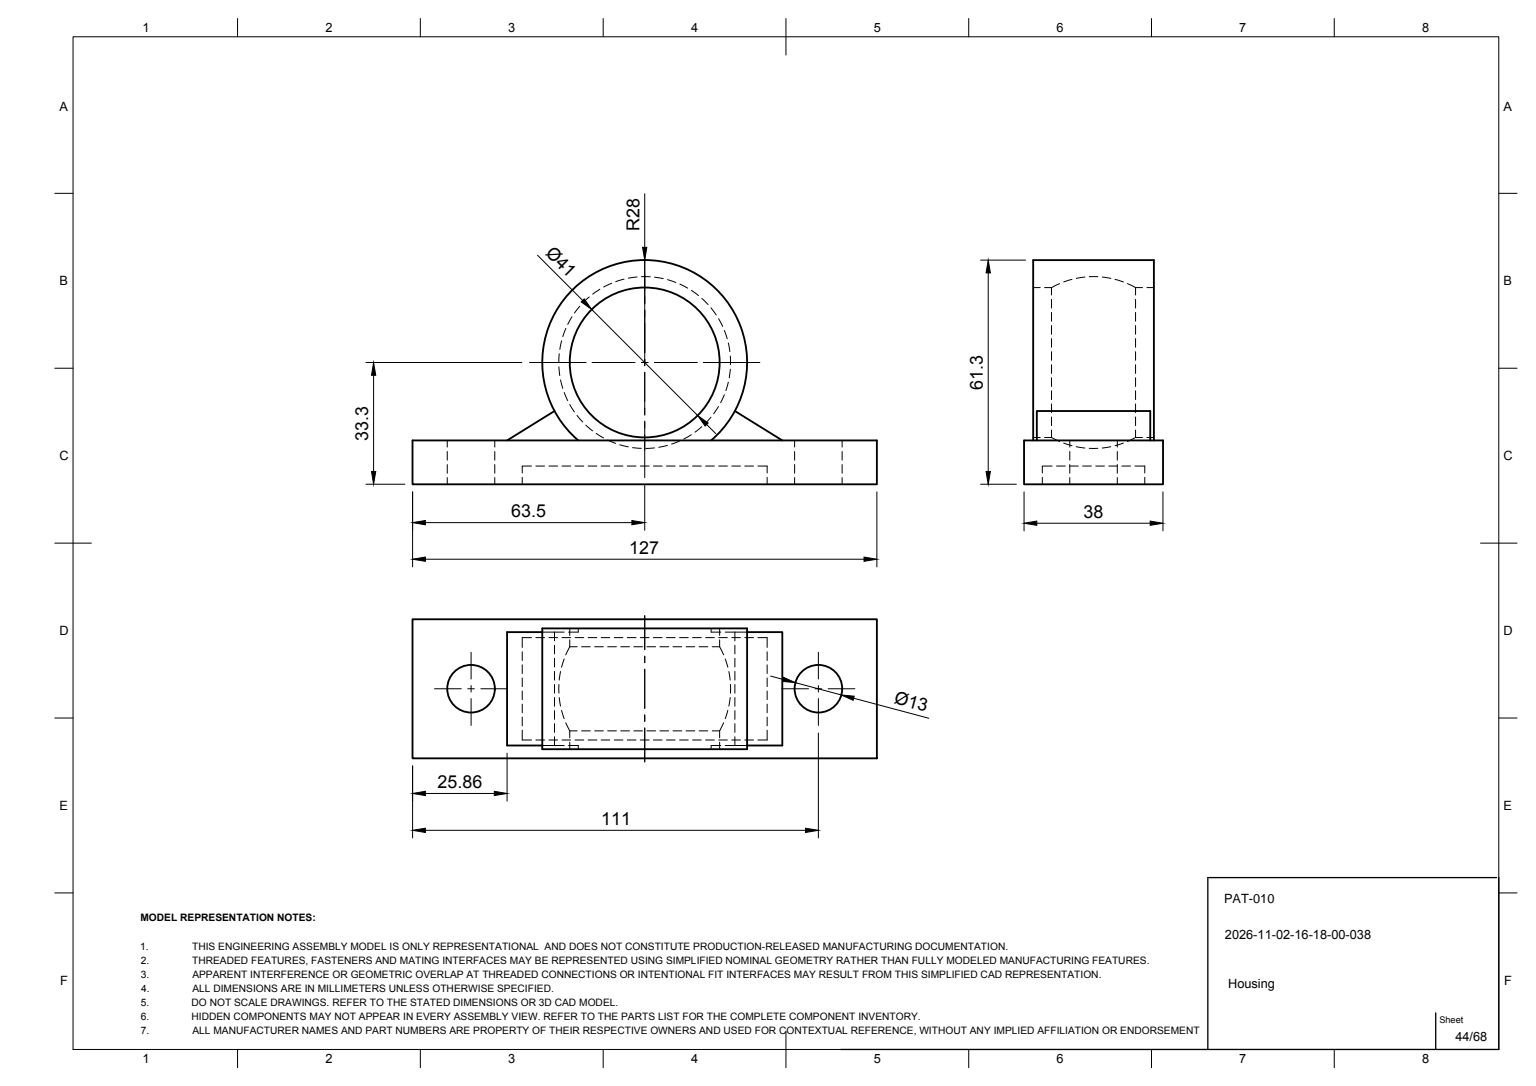
ISO-10303-21;
HEADER;
/* Generated by software containing ST-Developer
 * from STEP Tools, Inc. (www.steptools.com) 
 */

FILE_DESCRIPTION(
/* description */ ('Belt conveyor head drive unit'),
/* implementation_level */ '2;1');

FILE_NAME(
/* name */ 'Housing.step',
/* time_stamp */ '2026-10-28T03:26:19-07:00',
/* author */ (''),
/* organization */ (''),
/* preprocessor_version */ 'ST-DEVELOPER v20.2',
/* originating_system */ 'Autodesk Translation Framework v15.17.0.0',
/* authorisation */ '');

FILE_SCHEMA (('AUTOMOTIVE_DESIGN { 1 0 10303 214 3 1 1 }'));
ENDSEC;

DATA;
#10=MECHANICAL_DESIGN_GEOMETRIC_PRESENTATION_REPRESENTATION('',(#901),#27069);
#675=SPHERICAL_SURFACE('',#15515,2.35);
#748=SHAPE_REPRESENTATION_RELATIONSHIP('SRR','None',#27395,#817);
#817=ADVANCED_BREP_SHAPE_REPRESENTATION('',(#984),#27037);
#901=STYLED_ITEM('',(#27776),#984);
#984=MANIFOLD_SOLID_BREP('Body1',#13768);
#1172=FACE_BOUND('',#3033,.T.);
#1173=FACE_BOUND('',#3034,.T.);
#1174=FACE_BOUND('',#3042,.T.);
#1175=FACE_BOUND('',#3043,.T.);
#1176=FACE_BOUND('',#3044,.T.);
#1177=FACE_BOUND('',#3047,.T.);
#1178=FACE_BOUND('',#3049,.T.);
#1179=FACE_BOUND('',#3062,.T.);
#1180=FACE_BOUND('',#3063,.T.);
#1181=FACE_BOUND('',#3064,.T.);
#1493=PLANE('',#15517);
#1494=PLANE('',#15519);
#1495=PLANE('',#15521);
#1496=PLANE('',#15523);
#1497=PLANE('',#15524);
#1498=PLANE('',#15526);
#1499=PLANE('',#15527);
#1500=PLANE('',#15533);
#1501=PLANE('',#15534);
#1502=PLANE('',#15535);
#1503=PLANE('',#15536);
#1504=PLANE('',#15537);
#1505=PLANE('',#15538);
#1506=PLANE('',#15539);
#1507=PLANE('',#15544);
#1508=PLANE('',#15545);
#1509=PLANE('',#15546);
#1510=PLANE('',#15547);
#1511=PLANE('',#15548);
#2070=FACE_OUTER_BOUND('',#3030,.T.);
#2071=FACE_OUTER_BOUND('',#3031,.T.);
#2072=FACE_OUTER_BOUND('',#3032,.T.);
#2073=FACE_OUTER_BOUND('',#3035,.T.);
#2074=FACE_OUTER_BOUND('',#3036,.T.);
#2075=FACE_OUTER_BOUND('',#3037,.T.);
#2076=FACE_OUTER_BOUND('',#3038,.T.);
#2077=FACE_OUTER_BOUND('',#3039,.T.);
#2078=FACE_OUTER_BOUND('',#3040,.T.);
#2079=FACE_OUTER_BOUND('',#3041,.T.);
#2080=FACE_OUTER_BOUND('',#3045,.T.);
#2081=FACE_OUTER_BOUND('',#3046,.T.);
#2082=FACE_OUTER_BOUND('',#3048,.T.);
#2083=FACE_OUTER_BOUND('',#3050,.T.);
#2084=FACE_OUTER_BOUND('',#3051,.T.);
#2085=FACE_OUTER_BOUND('',#3052,.T.);
#2086=FACE_OUTER_BOUND('',#3053,.T.);
#2087=FACE_OUTER_BOUND('',#3054,.T.);
#2088=FACE_OUTER_BOUND('',#3055,.T.);
#2089=FACE_OUTER_BOUND('',#3056,.T.);
#2090=FACE_OUTER_BOUND('',#3057,.T.);
#2091=FACE_OUTER_BOUND('',#3058,.T.);
#2092=FACE_OUTER_BOUND('',#3059,.T.);
#2093=FACE_OUTER_BOUND('',#3060,.T.);
#2094=FACE_OUTER_BOUND('',#3061,.T.);
#3030=EDGE_LOOP('',(#10816,#10817,#10818,#10819));
#3031=EDGE_LOOP('',(#10820,#10821,#10822,#10823));
#3032=EDGE_LOOP('',(#10824,#10825));
#3033=EDGE_LOOP('',(#10826));
#3034=EDGE_LOOP('',(#10827));
#3035=EDGE_LOOP('',(#10828,#10829,#10830));
#3036=EDGE_LOOP('',(#10831,#10832,#10833));
#3037=EDGE_LOOP('',(#10834,#10835,#10836));
#3038=EDGE_LOOP('',(#10837,#10838,#10839,#10840));
#3039=EDGE_LOOP('',(#10841,#10842,#10843));
#3040=EDGE_LOOP('',(#10844,#10845,#10846,#10847));
#3041=EDGE_LOOP('',(#10848,#10849,#10850,#10851));
#3042=EDGE_LOOP('',(#10852));
#3043=EDGE_LOOP('',(#10853));
#3044=EDGE_LOOP('',(#10854,#10855,#10856,#10857,#10858,#10859,#10860,#10861,
#10862,#10863,#10864,#10865));
#3045=EDGE_LOOP('',(#10866,#10867,#10868,#10869,#10870,#10871,#10872,#10873,
#10874,#10875,#10876,#10877));
#3046=EDGE_LOOP('',(#10878,#10879));
#3047=EDGE_LOOP('',(#10880));
#3048=EDGE_LOOP('',(#10881,#10882));
#3049=EDGE_LOOP('',(#10883));
#3050=EDGE_LOOP('',(#10884,#10885,#10886,#10887));
#3051=EDGE_LOOP('',(#10888,#10889,#10890,#10891));
#3052=EDGE_LOOP('',(#10892,#10893,#10894,#10895));
#3053=EDGE_LOOP('',(#10896,#10897,#10898,#10899));
#3054=EDGE_LOOP('',(#10900,#10901,#10902,#10903));
#3055=EDGE_LOOP('',(#10904,#10905,#10906,#10907));
#3056=EDGE_LOOP('',(#10908,#10909,#10910,#10911));
#3057=EDGE_LOOP('',(#10912,#10913,#10914,#10915));
#3058=EDGE_LOOP('',(#10916,#10917,#10918,#10919));
#3059=EDGE_LOOP('',(#10920,#10921,#10922,#10923));
#3060=EDGE_LOOP('',(#10924,#10925,#10926,#10927));
#3061=EDGE_LOOP('',(#10928,#10929,#10930,#10931));
#3062=EDGE_LOOP('',(#10932,#10933,#10934,#10935));
#3063=EDGE_LOOP('',(#10936));
#3064=EDGE_LOOP('',(#10937));
#3940=LINE('',#23661,#4732);
#3941=LINE('',#23667,#4733);
#3942=LINE('',#23676,#4734);
#3943=LINE('',#23678,#4735);
#3944=LINE('',#23683,#4736);
#3945=LINE('',#23686,#4737);
#3946=LINE('',#23690,#4738);
#3947=LINE('',#23693,#4739);
#3948=LINE('',#23695,#4740);
#3949=LINE('',#23696,#4741);
#3950=LINE('',#23700,#4742);
#3951=LINE('',#23702,#4743);
#3952=LINE('',#23705,#4744);
#3953=LINE('',#23706,#4745);
#3954=LINE('',#23710,#4746);
#3955=LINE('',#23712,#4747);
#3956=LINE('',#23714,#4748);
#3957=LINE('',#23715,#4749);
#3958=LINE('',#23721,#4750);
#3959=LINE('',#23723,#4751);
#3960=LINE('',#23724,#4752);
#3961=LINE('',#23726,#4753);
#3962=LINE('',#23728,#4754);
#3963=LINE('',#23729,#4755);
#3964=LINE('',#23738,#4756);
#3965=LINE('',#23740,#4757);
#3966=LINE('',#23742,#4758);
#3967=LINE('',#23743,#4759);
#3968=LINE('',#23746,#4760);
#3969=LINE('',#23748,#4761);
#3970=LINE('',#23749,#4762);
#3971=LINE('',#23752,#4763);
#3972=LINE('',#23754,#4764);
#3973=LINE('',#23755,#4765);
#3974=LINE('',#23757,#4766);
#3975=LINE('',#23758,#4767);
#3976=LINE('',#23763,#4768);
#3977=LINE('',#23767,#4769);
#3978=LINE('',#23771,#4770);
#3979=LINE('',#23772,#4771);
#3980=LINE('',#23773,#4772);
#3981=LINE('',#23776,#4773);
#3982=LINE('',#23777,#4774);
#3983=LINE('',#23780,#4775);
#3984=LINE('',#23781,#4776);
#3985=LINE('',#23783,#4777);
#4732=VECTOR('',#18774,2.05);
#4733=VECTOR('',#18781,2.05);
#4734=VECTOR('',#18790,1.);
#4735=VECTOR('',#18791,1.);
#4736=VECTOR('',#18796,1.);
#4737=VECTOR('',#18799,1.);
#4738=VECTOR('',#18802,1.);
#4739=VECTOR('',#18805,1.);
#4740=VECTOR('',#18808,1.);
#4741=VECTOR('',#18809,1.);
#4742=VECTOR('',#18812,1.);
#4743=VECTOR('',#18813,1.);
#4744=VECTOR('',#18818,1.);
#4745=VECTOR('',#18819,1.);
#4746=VECTOR('',#18822,1.);
#4747=VECTOR('',#18823,1.);
#4748=VECTOR('',#18824,1.);
#4749=VECTOR('',#18825,1.);
#4750=VECTOR('',#18830,1.);
#4751=VECTOR('',#18831,1.);
#4752=VECTOR('',#18832,1.);
#4753=VECTOR('',#18833,1.);
#4754=VECTOR('',#18834,1.);
#4755=VECTOR('',#18835,1.);
#4756=VECTOR('',#18848,1.);
#4757=VECTOR('',#18849,1.);
#4758=VECTOR('',#18850,1.);
#4759=VECTOR('',#18851,1.);
#4760=VECTOR('',#18854,1.);
#4761=VECTOR('',#18855,1.);
#4762=VECTOR('',#18856,1.);
#4763=VECTOR('',#18859,1.);
#4764=VECTOR('',#18860,1.);
#4765=VECTOR('',#18861,1.);
#4766=VECTOR('',#18864,1.);
#4767=VECTOR('',#18865,1.);
#4768=VECTOR('',#18872,0.65);
#4769=VECTOR('',#18877,0.65);
#4770=VECTOR('',#18880,1.);
#4771=VECTOR('',#18881,1.);
#4772=VECTOR('',#18882,1.);
#4773=VECTOR('',#18885,1.);
#4774=VECTOR('',#18886,1.);
#4775=VECTOR('',#18889,1.);
#4776=VECTOR('',#18890,1.);
#4777=VECTOR('',#18893,1.);
#5537=CIRCLE('',#15510,2.05);
#5538=CIRCLE('',#15511,2.05);
#5539=CIRCLE('',#15513,2.05);
#5540=CIRCLE('',#15514,2.05);
#5541=CIRCLE('',#15516,2.35);
#5542=CIRCLE('',#15518,2.8);
#5543=CIRCLE('',#15520,2.8);
#5544=CIRCLE('',#15522,2.8);
#5545=CIRCLE('',#15525,2.8);
#5546=CIRCLE('',#15528,0.65);
#5547=CIRCLE('',#15529,0.65);
#5548=CIRCLE('',#15531,2.8);
#5549=CIRCLE('',#15532,2.8);
#5550=CIRCLE('',#15541,0.65);
#5551=CIRCLE('',#15543,0.65);
#6587=VERTEX_POINT('',#23658);
#6588=VERTEX_POINT('',#23660);
#6589=VERTEX_POINT('',#23664);
#6590=VERTEX_POINT('',#23666);
#6591=VERTEX_POINT('',#23670);
#6592=VERTEX_POINT('',#23671);
#6593=VERTEX_POINT('',#23674);
#6594=VERTEX_POINT('',#23675);
#6595=VERTEX_POINT('',#23677);
#6596=VERTEX_POINT('',#23681);
#6597=VERTEX_POINT('',#23682);
#6598=VERTEX_POINT('',#23684);
#6599=VERTEX_POINT('',#23688);
#6600=VERTEX_POINT('',#23689);
#6601=VERTEX_POINT('',#23691);
#6602=VERTEX_POINT('',#23698);
#6603=VERTEX_POINT('',#23699);
#6604=VERTEX_POINT('',#23701);
#6605=VERTEX_POINT('',#23708);
#6606=VERTEX_POINT('',#23709);
#6607=VERTEX_POINT('',#23711);
#6608=VERTEX_POINT('',#23713);
#6609=VERTEX_POINT('',#23716);
#6610=VERTEX_POINT('',#23718);
#6611=VERTEX_POINT('',#23720);
#6612=VERTEX_POINT('',#23722);
#6613=VERTEX_POINT('',#23725);
#6614=VERTEX_POINT('',#23727);
#6615=VERTEX_POINT('',#23736);
#6616=VERTEX_POINT('',#23737);
#6617=VERTEX_POINT('',#23739);
#6618=VERTEX_POINT('',#23741);
#6619=VERTEX_POINT('',#23745);
#6620=VERTEX_POINT('',#23747);
#6621=VERTEX_POINT('',#23751);
#6622=VERTEX_POINT('',#23753);
#6623=VERTEX_POINT('',#23761);
#6624=VERTEX_POINT('',#23765);
#6625=VERTEX_POINT('',#23769);
#6626=VERTEX_POINT('',#23770);
#6627=VERTEX_POINT('',#23775);
#6628=VERTEX_POINT('',#23779);
#8100=EDGE_CURVE('',#6587,#6587,#5537,.T.);
#8101=EDGE_CURVE('',#6587,#6588,#3940,.T.);
#8102=EDGE_CURVE('',#6588,#6588,#5538,.T.);
#8103=EDGE_CURVE('',#6589,#6589,#5539,.T.);
#8104=EDGE_CURVE('',#6589,#6590,#3941,.T.);
#8105=EDGE_CURVE('',#6590,#6590,#5540,.T.);
#8106=EDGE_CURVE('',#6591,#6592,#5541,.T.);
#8107=EDGE_CURVE('',#6593,#6594,#3942,.T.);
#8108=EDGE_CURVE('',#6593,#6595,#3943,.T.);
#8109=EDGE_CURVE('',#6594,#6595,#5542,.T.);
#8110=EDGE_CURVE('',#6596,#6597,#3944,.T.);
#8111=EDGE_CURVE('',#6598,#6596,#5543,.T.);
#8112=EDGE_CURVE('',#6598,#6597,#3945,.T.);
#8113=EDGE_CURVE('',#6599,#6600,#3946,.T.);
#8114=EDGE_CURVE('',#6601,#6599,#5544,.T.);
#8115=EDGE_CURVE('',#6601,#6600,#3947,.T.);
#8116=EDGE_CURVE('',#6600,#6593,#3948,.T.);
#8117=EDGE_CURVE('',#6595,#6601,#3949,.T.);
#8118=EDGE_CURVE('',#6602,#6603,#3950,.T.);
#8119=EDGE_CURVE('',#6602,#6604,#3951,.T.);
#8120=EDGE_CURVE('',#6603,#6604,#5545,.T.);
#8121=EDGE_CURVE('',#6597,#6602,#3952,.T.);
#8122=EDGE_CURVE('',#6604,#6598,#3953,.T.);
#8123=EDGE_CURVE('',#6605,#6606,#3954,.T.);
#8124=EDGE_CURVE('',#6606,#6607,#3955,.T.);
#8125=EDGE_CURVE('',#6607,#6608,#3956,.T.);
#8126=EDGE_CURVE('',#6608,#6605,#3957,.T.);
#8127=EDGE_CURVE('',#6609,#6609,#5546,.T.);
#8128=EDGE_CURVE('',#6610,#6610,#5547,.T.);
#8129=EDGE_CURVE('',#6603,#6611,#3958,.T.);
#8130=EDGE_CURVE('',#6611,#6612,#3959,.T.);
#8131=EDGE_CURVE('',#6612,#6599,#3960,.T.);
#8132=EDGE_CURVE('',#6594,#6613,#3961,.T.);
#8133=EDGE_CURVE('',#6613,#6614,#3962,.T.);
#8134=EDGE_CURVE('',#6614,#6596,#3963,.T.);
#8135=EDGE_CURVE('',#6613,#6614,#5548,.T.);
#8136=EDGE_CURVE('',#6611,#6612,#5549,.T.);
#8137=EDGE_CURVE('',#6615,#6616,#3964,.T.);
#8138=EDGE_CURVE('',#6615,#6617,#3965,.T.);
#8139=EDGE_CURVE('',#6617,#6618,#3966,.T.);
#8140=EDGE_CURVE('',#6616,#6618,#3967,.T.);
#8141=EDGE_CURVE('',#6619,#6615,#3968,.T.);
#8142=EDGE_CURVE('',#6619,#6620,#3969,.T.);
#8143=EDGE_CURVE('',#6620,#6617,#3970,.T.);
#8144=EDGE_CURVE('',#6621,#6619,#3971,.T.);
#8145=EDGE_CURVE('',#6621,#6622,#3972,.T.);
#8146=EDGE_CURVE('',#6622,#6620,#3973,.T.);
#8147=EDGE_CURVE('',#6616,#6621,#3974,.T.);
#8148=EDGE_CURVE('',#6618,#6622,#3975,.T.);
#8149=EDGE_CURVE('',#6623,#6623,#5550,.T.);
#8150=EDGE_CURVE('',#6623,#6610,#3976,.T.);
#8151=EDGE_CURVE('',#6624,#6624,#5551,.T.);
#8152=EDGE_CURVE('',#6624,#6609,#3977,.T.);
#8153=EDGE_CURVE('',#6625,#6626,#3978,.T.);
#8154=EDGE_CURVE('',#6626,#6605,#3979,.T.);
#8155=EDGE_CURVE('',#6625,#6608,#3980,.T.);
#8156=EDGE_CURVE('',#6627,#6625,#3981,.T.);
#8157=EDGE_CURVE('',#6627,#6607,#3982,.T.);
#8158=EDGE_CURVE('',#6628,#6627,#3983,.T.);
#8159=EDGE_CURVE('',#6628,#6606,#3984,.T.);
#8160=EDGE_CURVE('',#6626,#6628,#3985,.T.);
#10816=ORIENTED_EDGE('',*,*,#8100,.F.);
#10817=ORIENTED_EDGE('',*,*,#8101,.T.);
#10818=ORIENTED_EDGE('',*,*,#8102,.F.);
#10819=ORIENTED_EDGE('',*,*,#8101,.F.);
#10820=ORIENTED_EDGE('',*,*,#8103,.F.);
#10821=ORIENTED_EDGE('',*,*,#8104,.T.);
#10822=ORIENTED_EDGE('',*,*,#8105,.F.);
#10823=ORIENTED_EDGE('',*,*,#8104,.F.);
#10824=ORIENTED_EDGE('',*,*,#8106,.T.);
#10825=ORIENTED_EDGE('',*,*,#8106,.F.);
#10826=ORIENTED_EDGE('',*,*,#8103,.T.);
#10827=ORIENTED_EDGE('',*,*,#8102,.T.);
#10828=ORIENTED_EDGE('',*,*,#8107,.F.);
#10829=ORIENTED_EDGE('',*,*,#8108,.T.);
#10830=ORIENTED_EDGE('',*,*,#8109,.F.);
#10831=ORIENTED_EDGE('',*,*,#8110,.F.);
#10832=ORIENTED_EDGE('',*,*,#8111,.F.);
#10833=ORIENTED_EDGE('',*,*,#8112,.T.);
#10834=ORIENTED_EDGE('',*,*,#8113,.F.);
#10835=ORIENTED_EDGE('',*,*,#8114,.F.);
#10836=ORIENTED_EDGE('',*,*,#8115,.T.);
#10837=ORIENTED_EDGE('',*,*,#8116,.F.);
#10838=ORIENTED_EDGE('',*,*,#8115,.F.);
#10839=ORIENTED_EDGE('',*,*,#8117,.F.);
#10840=ORIENTED_EDGE('',*,*,#8108,.F.);
#10841=ORIENTED_EDGE('',*,*,#8118,.F.);
#10842=ORIENTED_EDGE('',*,*,#8119,.T.);
#10843=ORIENTED_EDGE('',*,*,#8120,.F.);
#10844=ORIENTED_EDGE('',*,*,#8121,.F.);
#10845=ORIENTED_EDGE('',*,*,#8112,.F.);
#10846=ORIENTED_EDGE('',*,*,#8122,.F.);
#10847=ORIENTED_EDGE('',*,*,#8119,.F.);
#10848=ORIENTED_EDGE('',*,*,#8123,.T.);
#10849=ORIENTED_EDGE('',*,*,#8124,.T.);
#10850=ORIENTED_EDGE('',*,*,#8125,.T.);
#10851=ORIENTED_EDGE('',*,*,#8126,.T.);
#10852=ORIENTED_EDGE('',*,*,#8127,.T.);
#10853=ORIENTED_EDGE('',*,*,#8128,.T.);
#10854=ORIENTED_EDGE('',*,*,#8110,.T.);
#10855=ORIENTED_EDGE('',*,*,#8121,.T.);
#10856=ORIENTED_EDGE('',*,*,#8118,.T.);
#10857=ORIENTED_EDGE('',*,*,#8129,.T.);
#10858=ORIENTED_EDGE('',*,*,#8130,.T.);
#10859=ORIENTED_EDGE('',*,*,#8131,.T.);
#10860=ORIENTED_EDGE('',*,*,#8113,.T.);
#10861=ORIENTED_EDGE('',*,*,#8116,.T.);
#10862=ORIENTED_EDGE('',*,*,#8107,.T.);
#10863=ORIENTED_EDGE('',*,*,#8132,.T.);
#10864=ORIENTED_EDGE('',*,*,#8133,.T.);
#10865=ORIENTED_EDGE('',*,*,#8134,.T.);
#10866=ORIENTED_EDGE('',*,*,#8111,.T.);
#10867=ORIENTED_EDGE('',*,*,#8134,.F.);
#10868=ORIENTED_EDGE('',*,*,#8135,.F.);
#10869=ORIENTED_EDGE('',*,*,#8132,.F.);
#10870=ORIENTED_EDGE('',*,*,#8109,.T.);
#10871=ORIENTED_EDGE('',*,*,#8117,.T.);
#10872=ORIENTED_EDGE('',*,*,#8114,.T.);
#10873=ORIENTED_EDGE('',*,*,#8131,.F.);
#10874=ORIENTED_EDGE('',*,*,#8136,.F.);
#10875=ORIENTED_EDGE('',*,*,#8129,.F.);
#10876=ORIENTED_EDGE('',*,*,#8120,.T.);
#10877=ORIENTED_EDGE('',*,*,#8122,.T.);
#10878=ORIENTED_EDGE('',*,*,#8130,.F.);
#10879=ORIENTED_EDGE('',*,*,#8136,.T.);
#10880=ORIENTED_EDGE('',*,*,#8100,.T.);
#10881=ORIENTED_EDGE('',*,*,#8133,.F.);
#10882=ORIENTED_EDGE('',*,*,#8135,.T.);
#10883=ORIENTED_EDGE('',*,*,#8105,.T.);
#10884=ORIENTED_EDGE('',*,*,#8137,.F.);
#10885=ORIENTED_EDGE('',*,*,#8138,.T.);
#10886=ORIENTED_EDGE('',*,*,#8139,.T.);
#10887=ORIENTED_EDGE('',*,*,#8140,.F.);
#10888=ORIENTED_EDGE('',*,*,#8141,.F.);
#10889=ORIENTED_EDGE('',*,*,#8142,.T.);
#10890=ORIENTED_EDGE('',*,*,#8143,.T.);
#10891=ORIENTED_EDGE('',*,*,#8138,.F.);
#10892=ORIENTED_EDGE('',*,*,#8144,.F.);
#10893=ORIENTED_EDGE('',*,*,#8145,.T.);
#10894=ORIENTED_EDGE('',*,*,#8146,.T.);
#10895=ORIENTED_EDGE('',*,*,#8142,.F.);
#10896=ORIENTED_EDGE('',*,*,#8147,.F.);
#10897=ORIENTED_EDGE('',*,*,#8140,.T.);
#10898=ORIENTED_EDGE('',*,*,#8148,.T.);
#10899=ORIENTED_EDGE('',*,*,#8145,.F.);
#10900=ORIENTED_EDGE('',*,*,#8148,.F.);
#10901=ORIENTED_EDGE('',*,*,#8139,.F.);
#10902=ORIENTED_EDGE('',*,*,#8143,.F.);
#10903=ORIENTED_EDGE('',*,*,#8146,.F.);
#10904=ORIENTED_EDGE('',*,*,#8149,.F.);
#10905=ORIENTED_EDGE('',*,*,#8150,.T.);
#10906=ORIENTED_EDGE('',*,*,#8128,.F.);
#10907=ORIENTED_EDGE('',*,*,#8150,.F.);
#10908=ORIENTED_EDGE('',*,*,#8151,.F.);
#10909=ORIENTED_EDGE('',*,*,#8152,.T.);
#10910=ORIENTED_EDGE('',*,*,#8127,.F.);
#10911=ORIENTED_EDGE('',*,*,#8152,.F.);
#10912=ORIENTED_EDGE('',*,*,#8153,.T.);
#10913=ORIENTED_EDGE('',*,*,#8154,.T.);
#10914=ORIENTED_EDGE('',*,*,#8126,.F.);
#10915=ORIENTED_EDGE('',*,*,#8155,.F.);
#10916=ORIENTED_EDGE('',*,*,#8156,.T.);
#10917=ORIENTED_EDGE('',*,*,#8155,.T.);
#10918=ORIENTED_EDGE('',*,*,#8125,.F.);
#10919=ORIENTED_EDGE('',*,*,#8157,.F.);
#10920=ORIENTED_EDGE('',*,*,#8158,.T.);
#10921=ORIENTED_EDGE('',*,*,#8157,.T.);
#10922=ORIENTED_EDGE('',*,*,#8124,.F.);
#10923=ORIENTED_EDGE('',*,*,#8159,.F.);
#10924=ORIENTED_EDGE('',*,*,#8160,.T.);
#10925=ORIENTED_EDGE('',*,*,#8159,.T.);
#10926=ORIENTED_EDGE('',*,*,#8123,.F.);
#10927=ORIENTED_EDGE('',*,*,#8154,.F.);
#10928=ORIENTED_EDGE('',*,*,#8160,.F.);
#10929=ORIENTED_EDGE('',*,*,#8153,.F.);
#10930=ORIENTED_EDGE('',*,*,#8156,.F.);
#10931=ORIENTED_EDGE('',*,*,#8158,.F.);
#10932=ORIENTED_EDGE('',*,*,#8137,.T.);
#10933=ORIENTED_EDGE('',*,*,#8147,.T.);
#10934=ORIENTED_EDGE('',*,*,#8144,.T.);
#10935=ORIENTED_EDGE('',*,*,#8141,.T.);
#10936=ORIENTED_EDGE('',*,*,#8149,.T.);
#10937=ORIENTED_EDGE('',*,*,#8151,.T.);
#12703=CYLINDRICAL_SURFACE('',#15509,2.05);
#12704=CYLINDRICAL_SURFACE('',#15512,2.05);
#12705=CYLINDRICAL_SURFACE('',#15530,2.8);
#12706=CYLINDRICAL_SURFACE('',#15540,0.65);
#12707=CYLINDRICAL_SURFACE('',#15542,0.65);
#13349=ADVANCED_FACE('',(#2070),#12703,.F.);
#13350=ADVANCED_FACE('',(#2071),#12704,.F.);
#13351=ADVANCED_FACE('',(#2072,#1172,#1173),#675,.F.);
#13352=ADVANCED_FACE('',(#2073),#1493,.T.);
#13353=ADVANCED_FACE('',(#2074),#1494,.T.);
#13354=ADVANCED_FACE('',(#2075),#1495,.T.);
#13355=ADVANCED_FACE('',(#2076),#1496,.T.);
#13356=ADVANCED_FACE('',(#2077),#1497,.T.);
#13357=ADVANCED_FACE('',(#2078),#1498,.T.);
#13358=ADVANCED_FACE('',(#2079,#1174,#1175,#1176),#1499,.T.);
#13359=ADVANCED_FACE('',(#2080),#12705,.T.);
#13360=ADVANCED_FACE('',(#2081,#1177),#1500,.F.);
#13361=ADVANCED_FACE('',(#2082,#1178),#1501,.T.);
#13362=ADVANCED_FACE('',(#2083),#1502,.F.);
#13363=ADVANCED_FACE('',(#2084),#1503,.F.);
#13364=ADVANCED_FACE('',(#2085),#1504,.F.);
#13365=ADVANCED_FACE('',(#2086),#1505,.F.);
#13366=ADVANCED_FACE('',(#2087),#1506,.F.);
#13367=ADVANCED_FACE('',(#2088),#12706,.F.);
#13368=ADVANCED_FACE('',(#2089),#12707,.F.);
#13369=ADVANCED_FACE('',(#2090),#1507,.T.);
#13370=ADVANCED_FACE('',(#2091),#1508,.T.);
#13371=ADVANCED_FACE('',(#2092),#1509,.T.);
#13372=ADVANCED_FACE('',(#2093),#1510,.T.);
#13373=ADVANCED_FACE('',(#2094,#1179,#1180,#1181),#1511,.F.);
#13768=CLOSED_SHELL('',(#13349,#13350,#13351,#13352,#13353,#13354,#13355,
#13356,#13357,#13358,#13359,#13360,#13361,#13362,#13363,#13364,#13365,#13366,
#13367,#13368,#13369,#13370,#13371,#13372,#13373));
#15508=AXIS2_PLACEMENT_3D('',#23656,#18768,#18769);
#15509=AXIS2_PLACEMENT_3D('',#23657,#18770,#18771);
#15510=AXIS2_PLACEMENT_3D('',#23659,#18772,#18773);
#15511=AXIS2_PLACEMENT_3D('',#23662,#18775,#18776);
#15512=AXIS2_PLACEMENT_3D('',#23663,#18777,#18778);
#15513=AXIS2_PLACEMENT_3D('',#23665,#18779,#18780);
#15514=AXIS2_PLACEMENT_3D('',#23668,#18782,#18783);
#15515=AXIS2_PLACEMENT_3D('',#23669,#18784,#18785);
#15516=AXIS2_PLACEMENT_3D('',#23672,#18786,#18787);
#15517=AXIS2_PLACEMENT_3D('',#23673,#18788,#18789);
#15518=AXIS2_PLACEMENT_3D('',#23679,#18792,#18793);
#15519=AXIS2_PLACEMENT_3D('',#23680,#18794,#18795);
#15520=AXIS2_PLACEMENT_3D('',#23685,#18797,#18798);
#15521=AXIS2_PLACEMENT_3D('',#23687,#18800,#18801);
#15522=AXIS2_PLACEMENT_3D('',#23692,#18803,#18804);
#15523=AXIS2_PLACEMENT_3D('',#23694,#18806,#18807);
#15524=AXIS2_PLACEMENT_3D('',#23697,#18810,#18811);
#15525=AXIS2_PLACEMENT_3D('',#23703,#18814,#18815);
#15526=AXIS2_PLACEMENT_3D('',#23704,#18816,#18817);
#15527=AXIS2_PLACEMENT_3D('',#23707,#18820,#18821);
#15528=AXIS2_PLACEMENT_3D('',#23717,#18826,#18827);
#15529=AXIS2_PLACEMENT_3D('',#23719,#18828,#18829);
#15530=AXIS2_PLACEMENT_3D('',#23730,#18836,#18837);
#15531=AXIS2_PLACEMENT_3D('',#23731,#18838,#18839);
#15532=AXIS2_PLACEMENT_3D('',#23732,#18840,#18841);
#15533=AXIS2_PLACEMENT_3D('',#23733,#18842,#18843);
#15534=AXIS2_PLACEMENT_3D('',#23734,#18844,#18845);
#15535=AXIS2_PLACEMENT_3D('',#23735,#18846,#18847);
#15536=AXIS2_PLACEMENT_3D('',#23744,#18852,#18853);
#15537=AXIS2_PLACEMENT_3D('',#23750,#18857,#18858);
#15538=AXIS2_PLACEMENT_3D('',#23756,#18862,#18863);
#15539=AXIS2_PLACEMENT_3D('',#23759,#18866,#18867);
#15540=AXIS2_PLACEMENT_3D('',#23760,#18868,#18869);
#15541=AXIS2_PLACEMENT_3D('',#23762,#18870,#18871);
#15542=AXIS2_PLACEMENT_3D('',#23764,#18873,#18874);
#15543=AXIS2_PLACEMENT_3D('',#23766,#18875,#18876);
#15544=AXIS2_PLACEMENT_3D('',#23768,#18878,#18879);
#15545=AXIS2_PLACEMENT_3D('',#23774,#18883,#18884);
#15546=AXIS2_PLACEMENT_3D('',#23778,#18887,#18888);
#15547=AXIS2_PLACEMENT_3D('',#23782,#18891,#18892);
#15548=AXIS2_PLACEMENT_3D('',#23784,#18894,#18895);
#18768=DIRECTION('axis',(0.,0.,1.));
#18769=DIRECTION('refdir',(1.,0.,0.));
#18770=DIRECTION('center_axis',(0.,1.,0.));
#18771=DIRECTION('ref_axis',(1.,0.,0.));
#18772=DIRECTION('center_axis',(0.,1.,0.));
#18773=DIRECTION('ref_axis',(1.,0.,0.));
#18774=DIRECTION('',(0.,1.,0.));
#18775=DIRECTION('center_axis',(0.,-1.,0.));
#18776=DIRECTION('ref_axis',(1.,0.,0.));
#18777=DIRECTION('center_axis',(0.,1.,0.));
#18778=DIRECTION('ref_axis',(1.,0.,0.));
#18779=DIRECTION('center_axis',(0.,1.,0.));
#18780=DIRECTION('ref_axis',(1.,0.,0.));
#18781=DIRECTION('',(0.,1.,0.));
#18782=DIRECTION('center_axis',(0.,-1.,0.));
#18783=DIRECTION('ref_axis',(1.,0.,0.));
#18784=DIRECTION('center_axis',(6.12323399573677E-17,0.,1.));
#18785=DIRECTION('ref_axis',(1.,0.,0.));
#18786=DIRECTION('center_axis',(-1.22464679914735E-16,1.,0.));
#18787=DIRECTION('ref_axis',(-1.,-1.22464679914735E-16,0.));
#18788=DIRECTION('center_axis',(0.,1.,0.));
#18789=DIRECTION('ref_axis',(0.,0.,1.));
#18790=DIRECTION('',(1.,0.,0.));
#18791=DIRECTION('',(0.850265146687862,0.,0.526354614616295));
#18792=DIRECTION('center_axis',(0.,1.,0.));
#18793=DIRECTION('ref_axis',(1.,0.,0.));
#18794=DIRECTION('center_axis',(0.,1.,0.));
#18795=DIRECTION('ref_axis',(0.,0.,1.));
#18796=DIRECTION('',(1.,0.,0.));
#18797=DIRECTION('center_axis',(0.,1.,0.));
#18798=DIRECTION('ref_axis',(1.,0.,0.));
#18799=DIRECTION('',(0.850265146687862,0.,-0.526354614616295));
#18800=DIRECTION('center_axis',(0.,-1.,0.));
#18801=DIRECTION('ref_axis',(0.,0.,-1.));
#18802=DIRECTION('',(-1.,0.,0.));
#18803=DIRECTION('center_axis',(0.,-1.,0.));
#18804=DIRECTION('ref_axis',(1.,0.,0.));
#18805=DIRECTION('',(-0.850265146687862,0.,-0.526354614616295));
#18806=DIRECTION('center_axis',(-0.526354614616295,0.,0.850265146687862));
#18807=DIRECTION('ref_axis',(0.850265146687862,0.,0.526354614616295));
#18808=DIRECTION('',(0.,1.,0.));
#18809=DIRECTION('',(0.,-1.,0.));
#18810=DIRECTION('center_axis',(0.,-1.,0.));
#18811=DIRECTION('ref_axis',(0.,0.,-1.));
#18812=DIRECTION('',(-1.,0.,0.));
#18813=DIRECTION('',(-0.850265146687862,0.,0.526354614616295));
#18814=DIRECTION('center_axis',(0.,-1.,0.));
#18815=DIRECTION('ref_axis',(1.,0.,0.));
#18816=DIRECTION('center_axis',(0.526354614616295,0.,0.850265146687862));
#18817=DIRECTION('ref_axis',(0.850265146687862,0.,-0.526354614616295));
#18818=DIRECTION('',(0.,-1.,0.));
#18819=DIRECTION('',(0.,1.,0.));
#18820=DIRECTION('center_axis',(0.,0.,1.));
#18821=DIRECTION('ref_axis',(1.,0.,0.));
#18822=DIRECTION('',(0.,-1.,0.));
#18823=DIRECTION('',(1.,0.,0.));
#18824=DIRECTION('',(0.,1.,0.));
#18825=DIRECTION('',(-1.,0.,0.));
#18826=DIRECTION('center_axis',(0.,0.,-1.));
#18827=DIRECTION('ref_axis',(1.,0.,0.));
#18828=DIRECTION('center_axis',(0.,0.,-1.));
#18829=DIRECTION('ref_axis',(1.,0.,0.));
#18830=DIRECTION('',(0.,-1.,0.));
#18831=DIRECTION('',(-1.,0.,0.));
#18832=DIRECTION('',(0.,1.,0.));
#18833=DIRECTION('',(0.,1.,0.));
#18834=DIRECTION('',(1.,0.,0.));
#18835=DIRECTION('',(0.,-1.,0.));
#18836=DIRECTION('center_axis',(0.,1.,0.));
#18837=DIRECTION('ref_axis',(6.12323399573677E-17,0.,1.));
#18838=DIRECTION('center_axis',(0.,1.,0.));
#18839=DIRECTION('ref_axis',(1.,0.,0.));
#18840=DIRECTION('center_axis',(0.,-1.,0.));
#18841=DIRECTION('ref_axis',(1.,0.,0.));
#18842=DIRECTION('center_axis',(0.,1.,0.));
#18843=DIRECTION('ref_axis',(1.,0.,0.));
#18844=DIRECTION('center_axis',(0.,1.,0.));
#18845=DIRECTION('ref_axis',(1.,0.,0.));
#18846=DIRECTION('center_axis',(0.,1.,0.));
#18847=DIRECTION('ref_axis',(-1.,0.,0.));
#18848=DIRECTION('',(-1.,0.,0.));
#18849=DIRECTION('',(0.,0.,1.));
#18850=DIRECTION('',(-1.,0.,0.));
#18851=DIRECTION('',(0.,0.,1.));
#18852=DIRECTION('center_axis',(1.,0.,0.));
#18853=DIRECTION('ref_axis',(0.,1.,0.));
#18854=DIRECTION('',(0.,1.,0.));
#18855=DIRECTION('',(0.,0.,1.));
#18856=DIRECTION('',(0.,1.,0.));
#18857=DIRECTION('center_axis',(0.,-1.,0.));
#18858=DIRECTION('ref_axis',(1.,0.,0.));
#18859=DIRECTION('',(1.,0.,0.));
#18860=DIRECTION('',(0.,0.,1.));
#18861=DIRECTION('',(1.,0.,0.));
#18862=DIRECTION('center_axis',(-1.,0.,0.));
#18863=DIRECTION('ref_axis',(0.,-1.,0.));
#18864=DIRECTION('',(0.,-1.,0.));
#18865=DIRECTION('',(0.,-1.,0.));
#18866=DIRECTION('center_axis',(0.,0.,1.));
#18867=DIRECTION('ref_axis',(1.,0.,0.));
#18868=DIRECTION('center_axis',(0.,0.,1.));
#18869=DIRECTION('ref_axis',(1.,0.,0.));
#18870=DIRECTION('center_axis',(0.,0.,1.));
#18871=DIRECTION('ref_axis',(1.,0.,0.));
#18872=DIRECTION('',(0.,0.,1.));
#18873=DIRECTION('center_axis',(0.,0.,1.));
#18874=DIRECTION('ref_axis',(1.,0.,0.));
#18875=DIRECTION('center_axis',(0.,0.,1.));
#18876=DIRECTION('ref_axis',(1.,0.,0.));
#18877=DIRECTION('',(0.,0.,1.));
#18878=DIRECTION('center_axis',(0.,1.,0.));
#18879=DIRECTION('ref_axis',(-1.,0.,0.));
#18880=DIRECTION('',(-1.,0.,0.));
#18881=DIRECTION('',(0.,0.,1.));
#18882=DIRECTION('',(0.,0.,1.));
#18883=DIRECTION('center_axis',(1.,0.,0.));
#18884=DIRECTION('ref_axis',(0.,1.,0.));
#18885=DIRECTION('',(0.,1.,0.));
#18886=DIRECTION('',(0.,0.,1.));
#18887=DIRECTION('center_axis',(0.,-1.,0.));
#18888=DIRECTION('ref_axis',(1.,0.,0.));
#18889=DIRECTION('',(1.,0.,0.));
#18890=DIRECTION('',(0.,0.,1.));
#18891=DIRECTION('center_axis',(-1.,0.,0.));
#18892=DIRECTION('ref_axis',(0.,-1.,0.));
#18893=DIRECTION('',(0.,-1.,0.));
#18894=DIRECTION('center_axis',(0.,0.,1.));
#18895=DIRECTION('ref_axis',(1.,0.,0.));
#23656=CARTESIAN_POINT('',(0.,0.,0.));
#23657=CARTESIAN_POINT('Origin',(0.,0.,0.));
#23658=CARTESIAN_POINT('',(-2.05,-1.65,2.51052593825207E-16));
#23659=CARTESIAN_POINT('Origin',(0.,-1.65,0.));
#23660=CARTESIAN_POINT('',(-2.05,-1.14891252930761,-2.51052593825207E-16));
#23661=CARTESIAN_POINT('',(-2.05,0.,2.51052593825207E-16));
#23662=CARTESIAN_POINT('Origin',(0.,-1.14891252930761,0.));
#23663=CARTESIAN_POINT('Origin',(0.,0.,0.));
#23664=CARTESIAN_POINT('',(-2.05,1.14891252930761,2.51052593825207E-16));
#23665=CARTESIAN_POINT('Origin',(0.,1.14891252930761,0.));
#23666=CARTESIAN_POINT('',(-2.05,1.65,-2.51052593825207E-16));
#23667=CARTESIAN_POINT('',(-2.05,0.,2.51052593825207E-16));
#23668=CARTESIAN_POINT('Origin',(0.,1.65,0.));
#23669=CARTESIAN_POINT('Origin',(0.,0.,0.));
#23670=CARTESIAN_POINT('',(-1.43895998899814E-16,-1.76221774462768E-32,
-2.35));
#23671=CARTESIAN_POINT('',(-1.43895998899814E-16,-1.76221774462768E-32,
2.35));
#23672=CARTESIAN_POINT('Origin',(0.,0.,0.));
#23673=CARTESIAN_POINT('Origin',(0.,1.55,-1.49));
#23674=CARTESIAN_POINT('',(-3.76384615384615,1.55,-2.13));
#23675=CARTESIAN_POINT('',(-1.81744325908679,1.55,-2.13));
#23676=CARTESIAN_POINT('',(0.,1.55,-2.13));
#23677=CARTESIAN_POINT('',(-2.46585583768694,1.55,-1.32648218523477));
#23678=CARTESIAN_POINT('',(-1.68,1.55,-0.84));
#23679=CARTESIAN_POINT('Origin',(0.,1.55,0.));
#23680=CARTESIAN_POINT('Origin',(0.,1.55,-1.49));
#23681=CARTESIAN_POINT('',(1.81744325908679,1.55,-2.13));
#23682=CARTESIAN_POINT('',(3.76384615384615,1.55,-2.13));
#23683=CARTESIAN_POINT('',(0.,1.55,-2.13));
#23684=CARTESIAN_POINT('',(2.46585583768694,1.55,-1.32648218523477));
#23685=CARTESIAN_POINT('Origin',(0.,1.55,0.));
#23686=CARTESIAN_POINT('',(3.78,1.55,-2.14));
#23687=CARTESIAN_POINT('Origin',(0.,-1.55,-1.49));
#23688=CARTESIAN_POINT('',(-1.81744325908679,-1.55,-2.13));
#23689=CARTESIAN_POINT('',(-3.76384615384615,-1.55,-2.13));
#23690=CARTESIAN_POINT('',(0.,-1.55,-2.13));
#23691=CARTESIAN_POINT('',(-2.46585583768694,-1.55,-1.32648218523477));
#23692=CARTESIAN_POINT('Origin',(0.,-1.55,0.));
#23693=CARTESIAN_POINT('',(-1.68,-1.55,-0.84));
#23694=CARTESIAN_POINT('Origin',(-3.78,0.,-2.14));
#23695=CARTESIAN_POINT('',(-3.76384615384615,0.,-2.13));
#23696=CARTESIAN_POINT('',(-2.46585583768694,0.,-1.32648218523477));
#23697=CARTESIAN_POINT('Origin',(0.,-1.55,-1.49));
#23698=CARTESIAN_POINT('',(3.76384615384615,-1.55,-2.13));
#23699=CARTESIAN_POINT('',(1.81744325908679,-1.55,-2.13));
#23700=CARTESIAN_POINT('',(0.,-1.55,-2.13));
#23701=CARTESIAN_POINT('',(2.46585583768694,-1.55,-1.32648218523477));
#23702=CARTESIAN_POINT('',(3.78,-1.55,-2.14));
#23703=CARTESIAN_POINT('Origin',(0.,-1.55,0.));
#23704=CARTESIAN_POINT('Origin',(1.68,0.,-0.84));
#23705=CARTESIAN_POINT('',(3.76384615384615,0.,-2.13));
#23706=CARTESIAN_POINT('',(2.46585583768694,0.,-1.32648218523477));
#23707=CARTESIAN_POINT('Origin',(0.,0.,-2.13));
#23708=CARTESIAN_POINT('',(-6.35,1.9,-2.13));
#23709=CARTESIAN_POINT('',(-6.35,-1.9,-2.13));
#23710=CARTESIAN_POINT('',(-6.35,1.9,-2.13));
#23711=CARTESIAN_POINT('',(6.35,-1.9,-2.13));
#23712=CARTESIAN_POINT('',(-6.35,-1.9,-2.13));
#23713=CARTESIAN_POINT('',(6.35,1.9,-2.13));
#23714=CARTESIAN_POINT('',(6.35,-1.9,-2.13));
#23715=CARTESIAN_POINT('',(6.35,1.9,-2.13));
#23716=CARTESIAN_POINT('',(4.1,7.9602041944578E-17,-2.13));
#23717=CARTESIAN_POINT('Origin',(4.75,0.,-2.13));
#23718=CARTESIAN_POINT('',(-5.4,7.9602041944578E-17,-2.13));
#23719=CARTESIAN_POINT('Origin',(-4.75,0.,-2.13));
#23720=CARTESIAN_POINT('',(1.81744325908679,-1.65,-2.13));
#23721=CARTESIAN_POINT('',(1.81744325908679,0.,-2.13));
#23722=CARTESIAN_POINT('',(-1.81744325908679,-1.65,-2.13));
#23723=CARTESIAN_POINT('',(0.,-1.65,-2.13));
#23724=CARTESIAN_POINT('',(-1.81744325908679,0.,-2.13));
#23725=CARTESIAN_POINT('',(-1.81744325908679,1.65,-2.13));
#23726=CARTESIAN_POINT('',(-1.81744325908679,0.,-2.13));
#23727=CARTESIAN_POINT('',(1.81744325908679,1.65,-2.13));
#23728=CARTESIAN_POINT('',(0.,1.65,-2.13));
#23729=CARTESIAN_POINT('',(1.81744325908679,0.,-2.13));
#23730=CARTESIAN_POINT('Origin',(0.,0.,0.));
#23731=CARTESIAN_POINT('Origin',(0.,1.65,0.));
#23732=CARTESIAN_POINT('Origin',(0.,-1.65,0.));
#23733=CARTESIAN_POINT('Origin',(0.,-1.65,0.));
#23734=CARTESIAN_POINT('Origin',(0.,1.65,0.));
#23735=CARTESIAN_POINT('Origin',(3.35,1.4,-3.33));
#23736=CARTESIAN_POINT('',(3.35,1.4,-3.33));
#23737=CARTESIAN_POINT('',(-3.35,1.4,-3.33));
#23738=CARTESIAN_POINT('',(1.675,1.4,-3.33));
#23739=CARTESIAN_POINT('',(3.35,1.4,-2.83));
#23740=CARTESIAN_POINT('',(3.35,1.4,-3.33));
#23741=CARTESIAN_POINT('',(-3.35,1.4,-2.83));
#23742=CARTESIAN_POINT('',(3.35,1.4,-2.83));
#23743=CARTESIAN_POINT('',(-3.35,1.4,-3.33));
#23744=CARTESIAN_POINT('Origin',(3.35,-1.4,-3.33));
#23745=CARTESIAN_POINT('',(3.35,-1.4,-3.33));
#23746=CARTESIAN_POINT('',(3.35,-0.7,-3.33));
#23747=CARTESIAN_POINT('',(3.35,-1.4,-2.83));
#23748=CARTESIAN_POINT('',(3.35,-1.4,-3.33));
#23749=CARTESIAN_POINT('',(3.35,-1.4,-2.83));
#23750=CARTESIAN_POINT('Origin',(-3.35,-1.4,-3.33));
#23751=CARTESIAN_POINT('',(-3.35,-1.4,-3.33));
#23752=CARTESIAN_POINT('',(-1.675,-1.4,-3.33));
#23753=CARTESIAN_POINT('',(-3.35,-1.4,-2.83));
#23754=CARTESIAN_POINT('',(-3.35,-1.4,-3.33));
#23755=CARTESIAN_POINT('',(-3.35,-1.4,-2.83));
#23756=CARTESIAN_POINT('Origin',(-3.35,1.4,-3.33));
#23757=CARTESIAN_POINT('',(-3.35,0.7,-3.33));
#23758=CARTESIAN_POINT('',(-3.35,1.4,-2.83));
#23759=CARTESIAN_POINT('Origin',(0.,0.,-2.83));
#23760=CARTESIAN_POINT('Origin',(-4.75,0.,-3.33));
#23761=CARTESIAN_POINT('',(-5.4,-7.9602041944578E-17,-3.33));
#23762=CARTESIAN_POINT('Origin',(-4.75,0.,-3.33));
#23763=CARTESIAN_POINT('',(-5.4,-7.9602041944578E-17,-3.33));
#23764=CARTESIAN_POINT('Origin',(4.75,0.,-3.33));
#23765=CARTESIAN_POINT('',(4.1,-7.9602041944578E-17,-3.33));
#23766=CARTESIAN_POINT('Origin',(4.75,0.,-3.33));
#23767=CARTESIAN_POINT('',(4.1,-7.9602041944578E-17,-3.33));
#23768=CARTESIAN_POINT('Origin',(6.35,1.9,-3.33));
#23769=CARTESIAN_POINT('',(6.35,1.9,-3.33));
#23770=CARTESIAN_POINT('',(-6.35,1.9,-3.33));
#23771=CARTESIAN_POINT('',(6.35,1.9,-3.33));
#23772=CARTESIAN_POINT('',(-6.35,1.9,-3.33));
#23773=CARTESIAN_POINT('',(6.35,1.9,-3.33));
#23774=CARTESIAN_POINT('Origin',(6.35,-1.9,-3.33));
#23775=CARTESIAN_POINT('',(6.35,-1.9,-3.33));
#23776=CARTESIAN_POINT('',(6.35,-1.9,-3.33));
#23777=CARTESIAN_POINT('',(6.35,-1.9,-3.33));
#23778=CARTESIAN_POINT('Origin',(-6.35,-1.9,-3.33));
#23779=CARTESIAN_POINT('',(-6.35,-1.9,-3.33));
#23780=CARTESIAN_POINT('',(-6.35,-1.9,-3.33));
#23781=CARTESIAN_POINT('',(-6.35,-1.9,-3.33));
#23782=CARTESIAN_POINT('Origin',(-6.35,1.9,-3.33));
#23783=CARTESIAN_POINT('',(-6.35,1.9,-3.33));
#23784=CARTESIAN_POINT('Origin',(0.,0.,-3.33));
#26960=UNCERTAINTY_MEASURE_WITH_UNIT(LENGTH_MEASURE(0.001),#27070,
'DISTANCE_ACCURACY_VALUE',
'Maximum model space distance between geometric entities at asserted c
onnectivities');
#26992=UNCERTAINTY_MEASURE_WITH_UNIT(LENGTH_MEASURE(0.001),#27070,
'DISTANCE_ACCURACY_VALUE',
'Maximum model space distance between geometric entities at asserted c
onnectivities');
#27037=(
GEOMETRIC_REPRESENTATION_CONTEXT(3)
GLOBAL_UNCERTAINTY_ASSIGNED_CONTEXT((#26960))
GLOBAL_UNIT_ASSIGNED_CONTEXT((#27070,#27072,#27073))
REPRESENTATION_CONTEXT('','3D')
);
#27069=(
GEOMETRIC_REPRESENTATION_CONTEXT(3)
GLOBAL_UNCERTAINTY_ASSIGNED_CONTEXT((#26992))
GLOBAL_UNIT_ASSIGNED_CONTEXT((#27070,#27072,#27073))
REPRESENTATION_CONTEXT('','3D')
);
#27070=(
LENGTH_UNIT()
NAMED_UNIT(*)
SI_UNIT(.CENTI.,.METRE.)
);
#27072=(
NAMED_UNIT(*)
PLANE_ANGLE_UNIT()
SI_UNIT($,.RADIAN.)
);
#27073=(
NAMED_UNIT(*)
SI_UNIT($,.STERADIAN.)
SOLID_ANGLE_UNIT()
);
#27118=SHAPE_DEFINITION_REPRESENTATION(#27204,#27395);
#27204=PRODUCT_DEFINITION_SHAPE('',$,#27472);
#27395=SHAPE_REPRESENTATION('',(#15508),#27037);
#27427=PRODUCT_DEFINITION_CONTEXT('part definition',#27657,'design');
#27472=PRODUCT_DEFINITION('Housing','Housing',#27548,#27427);
#27548=PRODUCT_DEFINITION_FORMATION('',$,#27703);
#27657=APPLICATION_CONTEXT(
'Core Data for Automotive Mechanical Design Process');
#27658=PRODUCT_CONTEXT('part definition',#27657,'mechanical');
#27703=PRODUCT('Housing','Housing','Housing',(#27658));
#27770=COLOUR_RGB('Dark Blue',0.08,0.2,0.34);
#27771=FILL_AREA_STYLE_COLOUR('',#27770);
#27772=FILL_AREA_STYLE('',(#27771));
#27773=SURFACE_STYLE_FILL_AREA(#27772);
#27774=SURFACE_SIDE_STYLE('',(#27773));
#27775=SURFACE_STYLE_USAGE(.BOTH.,#27774);
#27776=PRESENTATION_STYLE_ASSIGNMENT((#27775));
ENDSEC;
END-ISO-10303-21;
